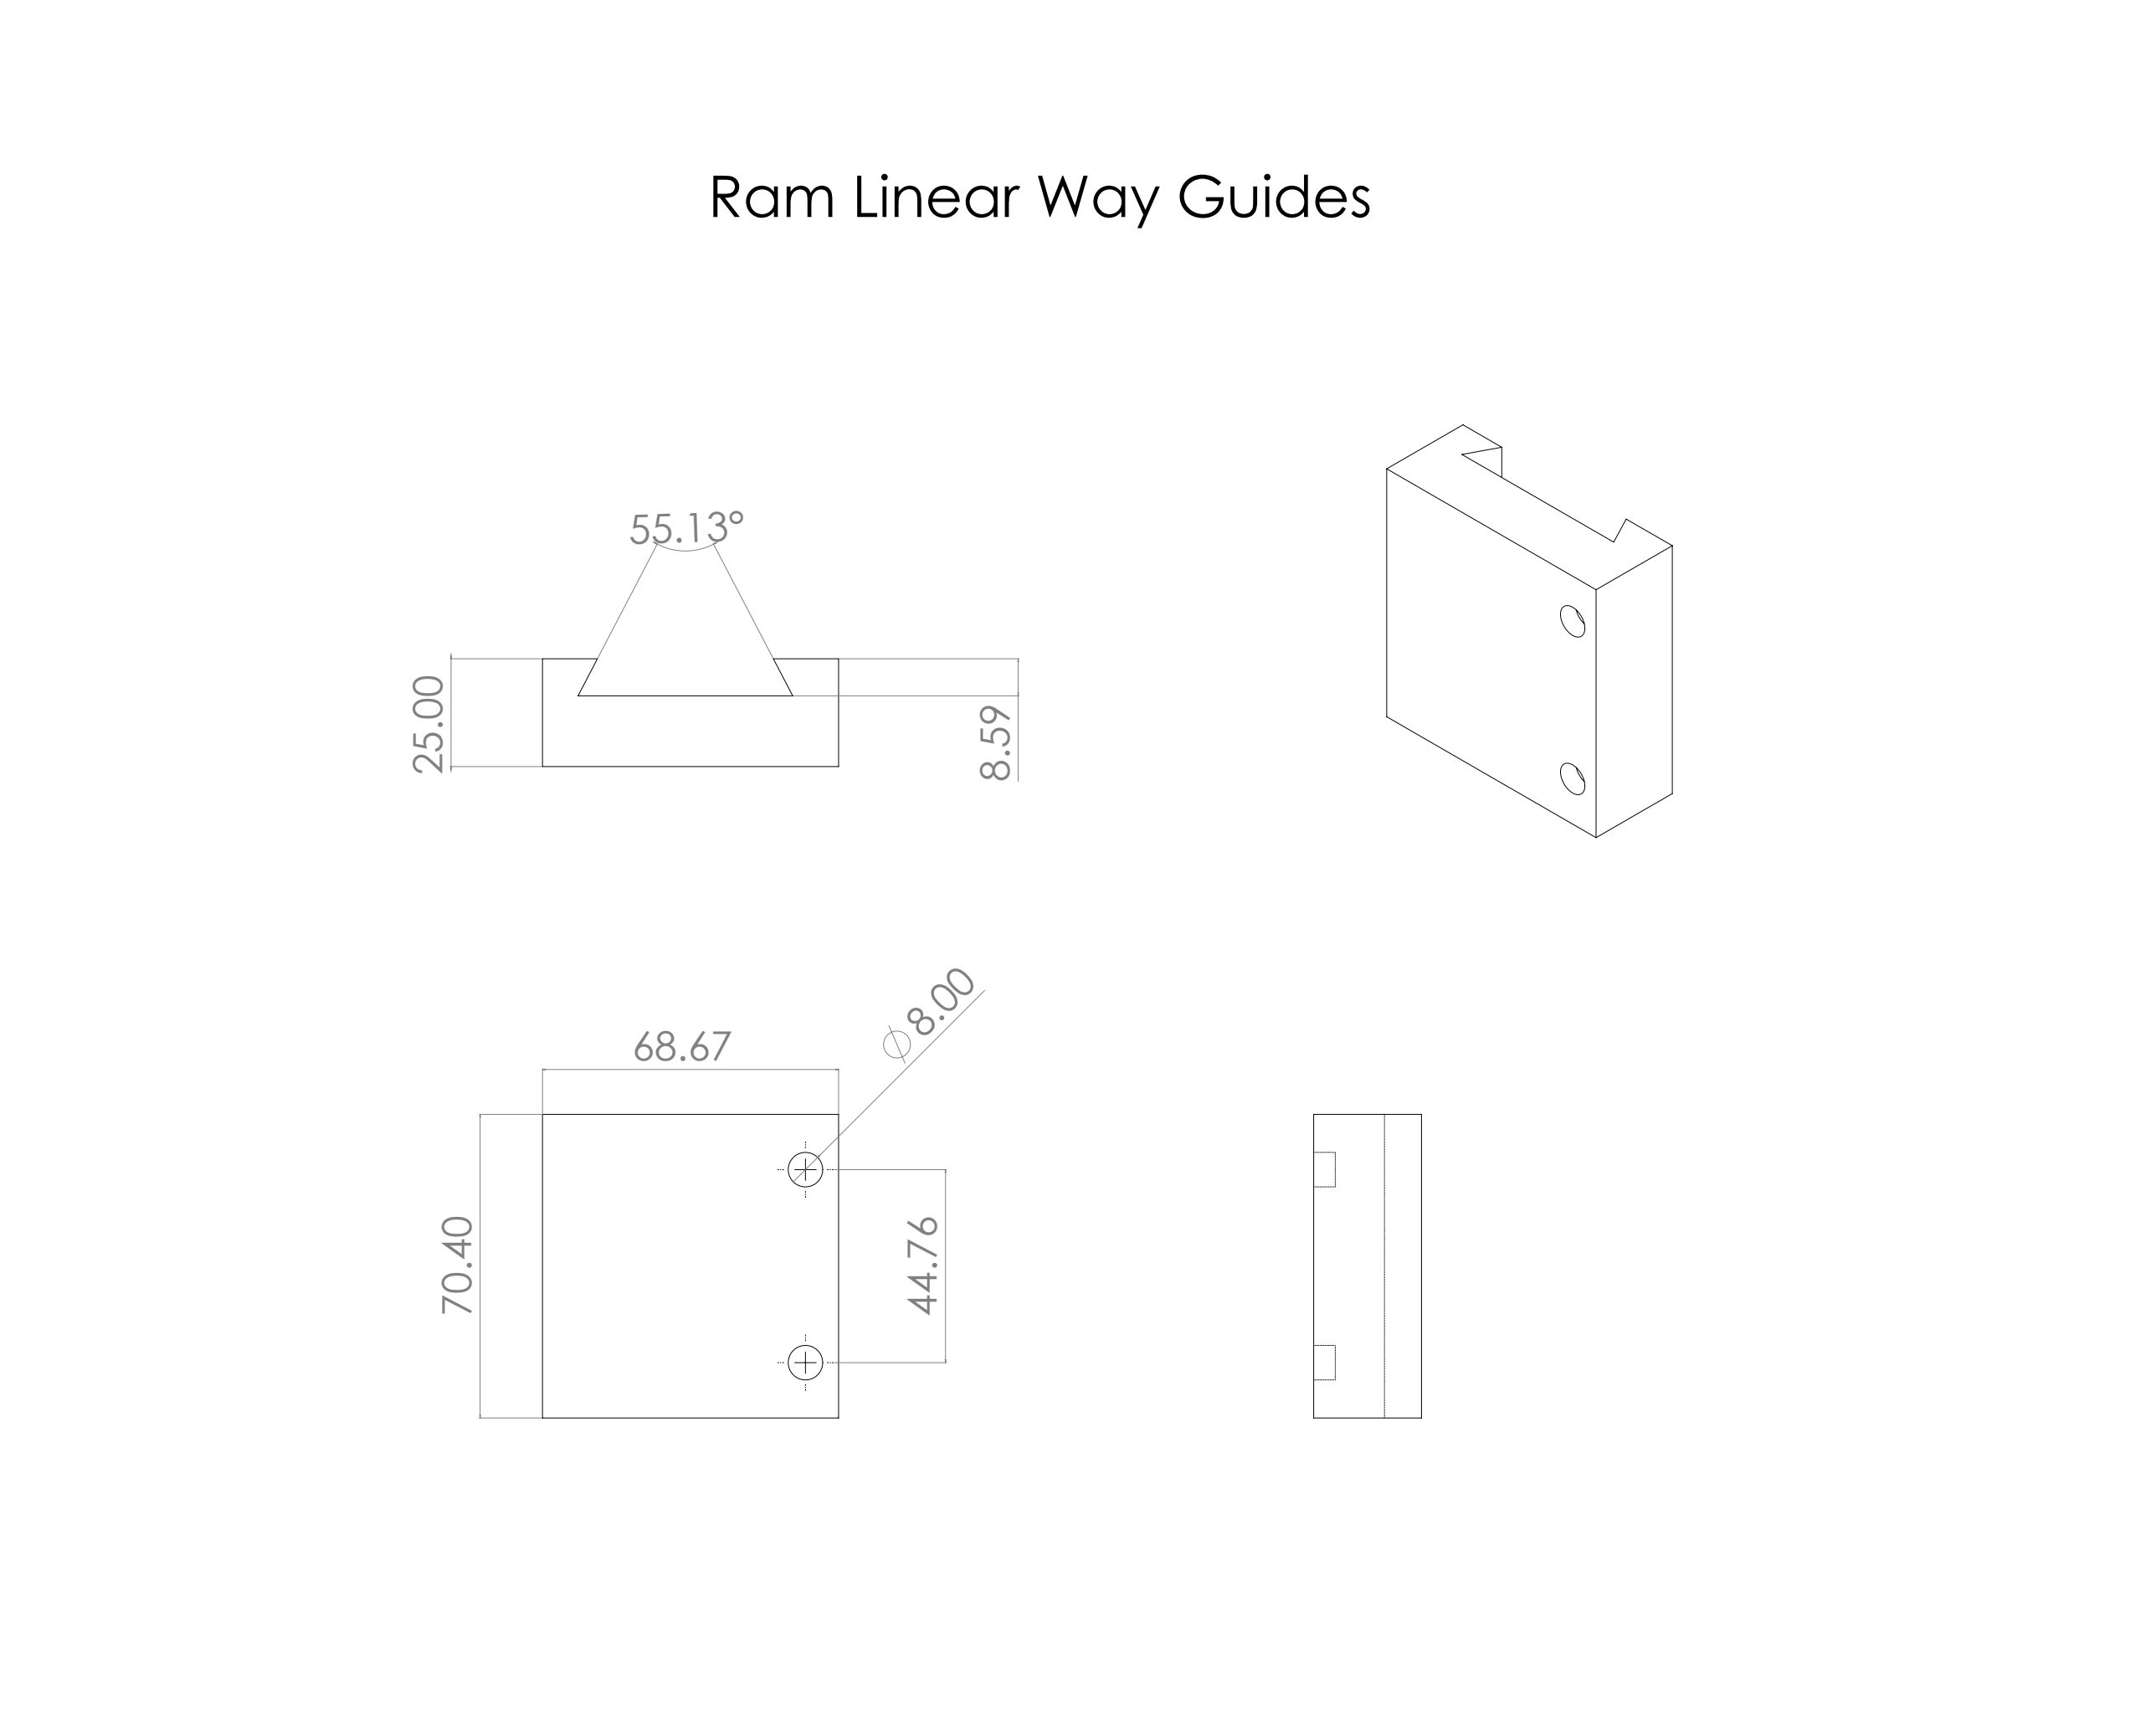
ISO-10303-21;
HEADER;
FILE_DESCRIPTION (('STEP AP214'),
    '1' );
FILE_NAME ('Ram Linear Way Guides.step',
    '2026-10-24T00:28:05',
    ( '' ),
    ( '' ),
    'SwSTEP 2.0',
    'SolidWorks 2025',
    '' );
FILE_SCHEMA (( 'AUTOMOTIVE_DESIGN' ));
ENDSEC;

DATA;
#156=CARTESIAN_POINT ( 'NONE',  ( -54.57497958038185004, 160.1716627696692683, 49.99999999999999289 ) ) ;
#191=ORIENTED_EDGE ( 'NONE', *, *, #19278, .F. ) ;
#197=DIRECTION ( 'NONE',  ( 0.000000000000000000, 0.000000000000000000, 1.000000000000000000 ) ) ;
#212=ORIENTED_EDGE ( 'NONE', *, *, #19326, .T. ) ;
#251=AXIS2_PLACEMENT_3D ( 'NONE', #16100, #3221, #14485 ) ;
#280=VECTOR ( 'NONE', #18343, 1000.000000000000000 ) ;
#332=DIRECTION ( 'NONE',  ( 0.000000000000000000, -0.000000000000000000, -1.000000000000000000 ) ) ;
#379=CARTESIAN_POINT ( 'NONE',  ( 6.416697501590670427, 172.9933428177121471, 45.00000000000000000 ) ) ;
#423=DIRECTION ( 'NONE',  ( 1.000000000000000000, 0.000000000000000000, -0.000000000000000000 ) ) ;
#438=DIRECTION ( 'NONE',  ( 0.000000000000000000, -1.000000000000000000, 0.000000000000000000 ) ) ;
#473=ORIENTED_EDGE ( 'NONE', *, *, #19536, .T. ) ;
#543=CARTESIAN_POINT ( 'NONE',  ( 10.41669750159067220, 217.7548513357008630, 45.00000000000000000 ) ) ;
#617=CARTESIAN_POINT ( 'NONE',  ( 6.416697501590670427, 172.9933428177121471, 49.99999999999999289 ) ) ;
#696=DIRECTION ( 'NONE',  ( 1.000000000000000000, 0.000000000000000000, 0.000000000000000000 ) ) ;
#718=( GEOMETRIC_REPRESENTATION_CONTEXT ( 3 ) GLOBAL_UNCERTAINTY_ASSIGNED_CONTEXT ( ( #1876 ) ) GLOBAL_UNIT_ASSIGNED_CONTEXT ( ( #11259, #6284, #3052 ) ) REPRESENTATION_CONTEXT ( 'NONE', 'WORKASPACE' ) );
#722=DIRECTION ( 'NONE',  ( 1.000000000000000000, 0.000000000000000000, 0.000000000000000000 ) ) ;
#751=CARTESIAN_POINT ( 'NONE',  ( 14.09825962131072785, 160.1716627696692683, 49.99999999999999289 ) ) ;
#808=CARTESIAN_POINT ( 'NONE',  ( 0.000000000000000000, 0.000000000000000000, 0.000000000000000000 ) ) ;
#884=PLANE ( 'NONE',  #19670 ) ;
#899=LINE ( 'NONE', #11030, #10091 ) ;
#918=PLANE ( 'NONE',  #7806 ) ;
#925=ORIENTED_EDGE ( 'NONE', *, *, #2214, .F. ) ;
#941=VECTOR ( 'NONE', #20908, 1000.000000000000000 ) ;
#965=PRODUCT_DEFINITION_SHAPE ( 'NONE', 'NONE',  #5449 ) ;
#976=ADVANCED_FACE ( 'NONE', ( #10029 ), #11976, .T. ) ;
#984=VERTEX_POINT ( 'NONE', #12082 ) ;
#1000=EDGE_CURVE ( 'NONE', #12300, #2829, #19044, .T. ) ;
#1005=DIRECTION ( 'NONE',  ( -1.000000000000000000, 0.000000000000000000, 0.000000000000000000 ) ) ;
#1044=DIRECTION ( 'NONE',  ( 0.000000000000000000, 0.000000000000000000, 1.000000000000000000 ) ) ;
#1053=CARTESIAN_POINT ( 'NONE',  ( -46.31968306282883674, 160.1716627696692683, 33.59072564020503648 ) ) ;
#1085=DIRECTION ( 'NONE',  ( -0.000000000000000000, -0.000000000000000000, 1.000000000000000000 ) ) ;
#1183=CARTESIAN_POINT ( 'NONE',  ( -41.83569717483972994, 303.6587712403113528, 25.00000000000000000 ) ) ;
#1274=VECTOR ( 'NONE', #21065, 1000.000000000000000 ) ;
#1308=CARTESIAN_POINT ( 'NONE',  ( 14.09825962131072785, 303.6587712403113528, 49.99999999999999289 ) ) ;
#1363=EDGE_LOOP ( 'NONE', ( #16478, #925, #12624, #3143 ) ) ;
#1437=CARTESIAN_POINT ( 'NONE',  ( 14.09825962131072785, 230.5765313837437418, 25.00000000000000000 ) ) ;
#1510=FACE_OUTER_BOUND ( 'NONE', #9710, .T. ) ;
#1527=LINE ( 'NONE', #9832, #3202 ) ;
#1544=CARTESIAN_POINT ( 'NONE',  ( 3.458603197740078627, 160.1716627696692683, 33.59072564020503648 ) ) ;
#1650=CARTESIAN_POINT ( 'NONE',  ( 6.416697501590670427, 217.7548513357008630, 49.99999999999999289 ) ) ;
#1668=LINE ( 'NONE', #2964, #11883 ) ;
#1698=ORIENTED_EDGE ( 'NONE', *, *, #13300, .F. ) ;
#1707=DIRECTION ( 'NONE',  ( 1.000000000000000000, 0.000000000000000000, 0.000000000000000000 ) ) ;
#1774=ORIENTED_EDGE ( 'NONE', *, *, #5730, .T. ) ;
#1777=LINE ( 'NONE', #19930, #14643 ) ;
#1778=ORIENTED_EDGE ( 'NONE', *, *, #18591, .F. ) ;
#1854=ORIENTED_EDGE ( 'NONE', *, *, #18917, .F. ) ;
#1856=ORIENTED_EDGE ( 'NONE', *, *, #19326, .F. ) ;
#1869=FACE_OUTER_BOUND ( 'NONE', #4529, .T. ) ;
#1876=UNCERTAINTY_MEASURE_WITH_UNIT (LENGTH_MEASURE( 1.000000000000000082E-05 ), #11259, 'distance_accuracy_value', 'NONE');
#1898=PLANE ( 'NONE',  #3083 ) ;
#2153=CYLINDRICAL_SURFACE ( 'NONE', #9746, 4.000000000000001776 ) ;
#2162=CIRCLE ( 'NONE', #7675, 4.000000000000001776 ) ;
#2214=EDGE_CURVE ( 'NONE', #17585, #2675, #8464, .T. ) ;
#2350=ORIENTED_EDGE ( 'NONE', *, *, #6167, .F. ) ;
#2386=DIRECTION ( 'NONE',  ( -0.000000000000000000, 0.000000000000000000, -1.000000000000000000 ) ) ;
#2394=DIRECTION ( 'NONE',  ( -1.000000000000000000, 0.000000000000000000, 0.000000000000000000 ) ) ;
#2419=DIRECTION ( 'NONE',  ( 0.000000000000000000, 0.000000000000000000, 1.000000000000000000 ) ) ;
#2535=VERTEX_POINT ( 'NONE', #10356 ) ;
#2564=AXIS2_PLACEMENT_3D ( 'NONE', #7882, #9824, #19676 ) ;
#2607=LINE ( 'NONE', #5840, #13238 ) ;
#2631=EDGE_CURVE ( 'NONE', #17585, #2829, #14280, .T. ) ;
#2675=VERTEX_POINT ( 'NONE', #20431 ) ;
#2704=DIRECTION ( 'NONE',  ( -1.000000000000000000, 0.000000000000000000, -0.000000000000000000 ) ) ;
#2721=VERTEX_POINT ( 'NONE', #751 ) ;
#2741=CARTESIAN_POINT ( 'NONE',  ( 2.416697501590669095, 172.9933428177121471, 49.99999999999999289 ) ) ;
#2751=ADVANCED_BREP_SHAPE_REPRESENTATION ( '', ( #19141, #12794 ), #718 ) ;
#2782=EDGE_LOOP ( 'NONE', ( #14261, #6010, #20550, #14725, #8206, #13930, #5554, #2865 ) ) ;
#2829=VERTEX_POINT ( 'NONE', #9157 ) ;
#2865=ORIENTED_EDGE ( 'NONE', *, *, #8030, .T. ) ;
#2910=VECTOR ( 'NONE', #1085, 1000.000000000000000 ) ;
#2964=CARTESIAN_POINT ( 'NONE',  ( 10.41669750159067220, 172.9933428177121471, 45.00000000000000000 ) ) ;
#3016=ORIENTED_EDGE ( 'NONE', *, *, #19278, .T. ) ;
#3052=( NAMED_UNIT ( * ) SI_UNIT ( $, .STERADIAN. ) SOLID_ANGLE_UNIT ( ) );
#3083=AXIS2_PLACEMENT_3D ( 'NONE', #379, #13571, #5328 ) ;
#3111=CARTESIAN_POINT ( 'NONE',  ( 2.416697501590669095, 217.7548513357008630, 49.99999999999999289 ) ) ;
#3121=ORIENTED_EDGE ( 'NONE', *, *, #16587, .F. ) ;
#3143=ORIENTED_EDGE ( 'NONE', *, *, #19941, .T. ) ;
#3150=EDGE_CURVE ( 'NONE', #16453, #6197, #1668, .T. ) ;
#3192=CARTESIAN_POINT ( 'NONE',  ( -54.57497958038185004, 230.5765313837437418, 49.99999999999999289 ) ) ;
#3198=EDGE_LOOP ( 'NONE', ( #21307, #15771, #9946, #212 ) ) ;
#3202=VECTOR ( 'NONE', #7993, 1000.000000000000000 ) ;
#3221=DIRECTION ( 'NONE',  ( -0.000000000000000000, -0.000000000000000000, 1.000000000000000000 ) ) ;
#3266=DIRECTION ( 'NONE',  ( -1.000000000000000000, 0.000000000000000000, 2.775557561562891844E-16 ) ) ;
#3364=CARTESIAN_POINT ( 'NONE',  ( -46.31968306282883674, 303.6587712403113528, 33.59072564020503648 ) ) ;
#3553=CARTESIAN_POINT ( 'NONE',  ( -41.83569717483972994, 303.6587712403113528, 25.00000000000000000 ) ) ;
#3716=EDGE_CURVE ( 'NONE', #6455, #20328, #899, .T. ) ;
#3717=VECTOR ( 'NONE', #20320, 1000.000000000000000 ) ;
#3750=ORIENTED_EDGE ( 'NONE', *, *, #16376, .T. ) ;
#3791=LINE ( 'NONE', #10277, #14282 ) ;
#3862=DIRECTION ( 'NONE',  ( 1.000000000000000000, 0.000000000000000000, 0.000000000000000000 ) ) ;
#3910=AXIS2_PLACEMENT_3D ( 'NONE', #617, #7181, #722 ) ;
#3927=EDGE_CURVE ( 'NONE', #20838, #9623, #1527, .T. ) ;
#3934=ORIENTED_EDGE ( 'NONE', *, *, #19941, .F. ) ;
#3969=CARTESIAN_POINT ( 'NONE',  ( -54.57497958038185715, 230.5765313837437418, 25.00000000000000000 ) ) ;
#4029=ADVANCED_FACE ( 'NONE', ( #20212 ), #2153, .F. ) ;
#4041=ORIENTED_EDGE ( 'NONE', *, *, #13300, .T. ) ;
#4089=CARTESIAN_POINT ( 'NONE',  ( 10.41669750159067220, 217.7548513357008630, 45.00000000000000000 ) ) ;
#4096=CARTESIAN_POINT ( 'NONE',  ( -54.57497958038185715, 303.6587712403113528, 25.00000000000000000 ) ) ;
#4162=DIRECTION ( 'NONE',  ( -0.000000000000000000, -0.000000000000000000, 1.000000000000000000 ) ) ;
#4200=AXIS2_PLACEMENT_3D ( 'NONE', #4096, #5933, #2704 ) ;
#4268=ORIENTED_EDGE ( 'NONE', *, *, #15151, .T. ) ;
#4273=CARTESIAN_POINT ( 'NONE',  ( -54.57497958038185715, 230.5765313837437418, 25.00000000000000000 ) ) ;
#4277=CARTESIAN_POINT ( 'NONE',  ( 14.09825962131072785, 160.1716627696692683, 25.00000000000000000 ) ) ;
#4340=ORIENTED_EDGE ( 'NONE', *, *, #20691, .T. ) ;
#4382=CARTESIAN_POINT ( 'NONE',  ( 6.416697501590670427, 172.9933428177121471, 45.00000000000000000 ) ) ;
#4436=CARTESIAN_POINT ( 'NONE',  ( -54.57497958038185004, 303.6587712403113528, 49.99999999999999289 ) ) ;
#4529=EDGE_LOOP ( 'NONE', ( #16668, #4268 ) ) ;
#4702=ORIENTED_EDGE ( 'NONE', *, *, #16376, .F. ) ;
#4717=( LENGTH_UNIT ( ) NAMED_UNIT ( * ) SI_UNIT ( .MILLI., .METRE. ) );
#4755=VERTEX_POINT ( 'NONE', #3192 ) ;
#4768=PLANE ( 'NONE',  #10337 ) ;
#4794=PLANE ( 'NONE',  #18083 ) ;
#4858=UNCERTAINTY_MEASURE_WITH_UNIT (LENGTH_MEASURE( 1.000000000000000082E-05 ), #4717, 'distance_accuracy_value', 'NONE');
#4865=DIRECTION ( 'NONE',  ( -1.000000000000000000, 0.000000000000000000, 0.000000000000000000 ) ) ;
#5079=CARTESIAN_POINT ( 'NONE',  ( 6.416697501590670427, 172.9933428177121471, 45.00000000000000000 ) ) ;
#5081=ORIENTED_EDGE ( 'NONE', *, *, #3716, .F. ) ;
#5099=PRODUCT_DEFINITION_CONTEXT ( 'detailed design', #20777, 'design' ) ;
#5197=DIRECTION ( 'NONE',  ( 0.000000000000000000, 0.000000000000000000, 1.000000000000000000 ) ) ;
#5267=VERTEX_POINT ( 'NONE', #2741 ) ;
#5287=CARTESIAN_POINT ( 'NONE',  ( -1.025382690249031503, 230.5765313837437418, 25.00000000000000000 ) ) ;
#5328=DIRECTION ( 'NONE',  ( -1.000000000000000000, 0.000000000000000000, 0.000000000000000000 ) ) ;
#5348=EDGE_LOOP ( 'NONE', ( #1856, #19473 ) ) ;
#5449=PRODUCT_DEFINITION ( 'UNKNOWN', '', #17987, #5099 ) ;
#5474=ORIENTED_EDGE ( 'NONE', *, *, #6268, .T. ) ;
#5482=DIRECTION ( 'NONE',  ( 0.8865057725575725689, 0.000000000000000000, 0.4627175328665443232 ) ) ;
#5514=PLANE ( 'NONE',  #18980 ) ;
#5528=ORIENTED_EDGE ( 'NONE', *, *, #11209, .T. ) ;
#5554=ORIENTED_EDGE ( 'NONE', *, *, #6229, .T. ) ;
#5582=ORIENTED_EDGE ( 'NONE', *, *, #17769, .T. ) ;
#5730=EDGE_CURVE ( 'NONE', #4755, #15709, #12562, .T. ) ;
#5819=EDGE_LOOP ( 'NONE', ( #17219, #13840, #8937, #1698 ) ) ;
#5840=CARTESIAN_POINT ( 'NONE',  ( -46.31968306282883674, 160.1716627696692683, 33.59072564020503648 ) ) ;
#5867=DIRECTION ( 'NONE',  ( -0.4627175328665442677, 0.000000000000000000, -0.8865057725575725689 ) ) ;
#5891=CYLINDRICAL_SURFACE ( 'NONE', #10934, 4.000000000000001776 ) ;
#5933=DIRECTION ( 'NONE',  ( 0.000000000000000000, 0.000000000000000000, -1.000000000000000000 ) ) ;
#5975=CIRCLE ( 'NONE', #19457, 4.000000000000001776 ) ;
#6010=ORIENTED_EDGE ( 'NONE', *, *, #7435, .T. ) ;
#6073=CARTESIAN_POINT ( 'NONE',  ( -54.57497958038185004, 230.5765313837437418, 49.99999999999999289 ) ) ;
#6113=ORIENTED_EDGE ( 'NONE', *, *, #13198, .T. ) ;
#6167=EDGE_CURVE ( 'NONE', #15709, #20838, #6614, .T. ) ;
#6197=VERTEX_POINT ( 'NONE', #6830 ) ;
#6214=CARTESIAN_POINT ( 'NONE',  ( -41.83569717483972994, 230.5765313837437418, 25.00000000000000000 ) ) ;
#6229=EDGE_CURVE ( 'NONE', #2535, #7734, #1777, .T. ) ;
#6268=EDGE_CURVE ( 'NONE', #2721, #15709, #7247, .T. ) ;
#6284=( NAMED_UNIT ( * ) PLANE_ANGLE_UNIT ( ) SI_UNIT ( $, .RADIAN. ) );
#6329=ORIENTED_EDGE ( 'NONE', *, *, #9299, .T. ) ;
#6411=FACE_OUTER_BOUND ( 'NONE', #7242, .T. ) ;
#6434=EDGE_CURVE ( 'NONE', #16453, #10176, #5975, .T. ) ;
#6455=VERTEX_POINT ( 'NONE', #5287 ) ;
#6493=DIRECTION ( 'NONE',  ( 1.000000000000000000, 0.000000000000000000, 0.000000000000000000 ) ) ;
#6525=VECTOR ( 'NONE', #14000, 1000.000000000000114 ) ;
#6614=LINE ( 'NONE', #156, #11507 ) ;
#6671=VECTOR ( 'NONE', #7077, 1000.000000000000000 ) ;
#6796=AXIS2_PLACEMENT_3D ( 'NONE', #10408, #18526, #13781 ) ;
#6817=CARTESIAN_POINT ( 'NONE',  ( 14.09825962131072785, 160.1716627696692683, 25.00000000000000000 ) ) ;
#6830=CARTESIAN_POINT ( 'NONE',  ( 10.41669750159067220, 172.9933428177121471, 49.99999999999999289 ) ) ;
#6996=ORIENTED_EDGE ( 'NONE', *, *, #17769, .F. ) ;
#6997=DIRECTION ( 'NONE',  ( 0.4627175328665442677, 0.000000000000000000, -0.8865057725575724579 ) ) ;
#7004=CARTESIAN_POINT ( 'NONE',  ( 20.42502041961813930, 230.5765313837437418, 60.00000000000000000 ) ) ;
#7006=VECTOR ( 'NONE', #19540, 1000.000000000000000 ) ;
#7021=CIRCLE ( 'NONE', #9096, 4.000000000000001776 ) ;
#7039=EDGE_LOOP ( 'NONE', ( #11206, #3750 ) ) ;
#7077=DIRECTION ( 'NONE',  ( 0.000000000000000000, -1.000000000000000000, 0.000000000000000000 ) ) ;
#7181=DIRECTION ( 'NONE',  ( 0.000000000000000000, 0.000000000000000000, 1.000000000000000000 ) ) ;
#7242=EDGE_LOOP ( 'NONE', ( #17088, #4041, #18357, #13154 ) ) ;
#7247=LINE ( 'NONE', #18826, #12567 ) ;
#7334=VERTEX_POINT ( 'NONE', #20095 ) ;
#7372=CARTESIAN_POINT ( 'NONE',  ( -41.83569717483972994, 160.1716627696692683, 25.00000000000000000 ) ) ;
#7435=EDGE_CURVE ( 'NONE', #4755, #984, #17066, .T. ) ;
#7478=CARTESIAN_POINT ( 'NONE',  ( 10.41669750159067220, 172.9933428177121471, 45.00000000000000000 ) ) ;
#7589=CARTESIAN_POINT ( 'NONE',  ( 3.458603197740078627, 160.1716627696692683, 33.59072564020503648 ) ) ;
#7660=FACE_OUTER_BOUND ( 'NONE', #12569, .T. ) ;
#7675=AXIS2_PLACEMENT_3D ( 'NONE', #19973, #197, #1707 ) ;
#7734=VERTEX_POINT ( 'NONE', #6214 ) ;
#7775=DIRECTION ( 'NONE',  ( 0.000000000000000000, -1.000000000000000000, 0.000000000000000000 ) ) ;
#7806=AXIS2_PLACEMENT_3D ( 'NONE', #14109, #14217, #20804 ) ;
#7847=AXIS2_PLACEMENT_3D ( 'NONE', #17108, #8867, #15067 ) ;
#7882=CARTESIAN_POINT ( 'NONE',  ( 6.416697501590670427, 217.7548513357008630, 45.00000000000000000 ) ) ;
#7993=DIRECTION ( 'NONE',  ( 1.000000000000000000, 0.000000000000000000, 0.000000000000000000 ) ) ;
#8030=EDGE_CURVE ( 'NONE', #7734, #8775, #15564, .T. ) ;
#8084=DIRECTION ( 'NONE',  ( -0.000000000000000000, -0.000000000000000000, 1.000000000000000000 ) ) ;
#8173=LINE ( 'NONE', #1183, #1274 ) ;
#8204=ORIENTED_EDGE ( 'NONE', *, *, #3927, .F. ) ;
#8206=ORIENTED_EDGE ( 'NONE', *, *, #3716, .T. ) ;
#8209=EDGE_LOOP ( 'NONE', ( #17696, #10470, #16403, #6996 ) ) ;
#8401=CIRCLE ( 'NONE', #3910, 4.000000000000001776 ) ;
#8464=CIRCLE ( 'NONE', #2564, 4.000000000000001776 ) ;
#8690=DIRECTION ( 'NONE',  ( 0.000000000000000000, -1.000000000000000000, 0.000000000000000000 ) ) ;
#8766=PLANE ( 'NONE',  #7847 ) ;
#8775=VERTEX_POINT ( 'NONE', #4273 ) ;
#8789=FACE_OUTER_BOUND ( 'NONE', #7039, .T. ) ;
#8867=DIRECTION ( 'NONE',  ( 0.000000000000000000, 0.000000000000000000, 1.000000000000000000 ) ) ;
#8937=ORIENTED_EDGE ( 'NONE', *, *, #20917, .F. ) ;
#9096=AXIS2_PLACEMENT_3D ( 'NONE', #1650, #10061, #6493 ) ;
#9130=CARTESIAN_POINT ( 'NONE',  ( 2.416697501590669095, 217.7548513357008630, 45.00000000000000000 ) ) ;
#9157=CARTESIAN_POINT ( 'NONE',  ( 10.41669750159067220, 217.7548513357008630, 49.99999999999999289 ) ) ;
#9175=ADVANCED_FACE ( 'NONE', ( #8789 ), #1898, .F. ) ;
#9241=CARTESIAN_POINT ( 'NONE',  ( 6.416697501590670427, 217.7548513357008630, 45.00000000000000000 ) ) ;
#9243=CARTESIAN_POINT ( 'NONE',  ( -54.57497958038185715, 160.1716627696692683, 25.00000000000000000 ) ) ;
#9269=VECTOR ( 'NONE', #16864, 1000.000000000000000 ) ;
#9292=FACE_OUTER_BOUND ( 'NONE', #5819, .T. ) ;
#9299=EDGE_CURVE ( 'NONE', #9623, #12668, #17652, .T. ) ;
#9377=LINE ( 'NONE', #15013, #7006 ) ;
#9383=FACE_OUTER_BOUND ( 'NONE', #17142, .T. ) ;
#9457=LINE ( 'NONE', #9130, #14990 ) ;
#9558=ADVANCED_FACE ( 'NONE', ( #16465 ), #4768, .T. ) ;
#9574=CIRCLE ( 'NONE', #12344, 4.000000000000001776 ) ;
#9623=VERTEX_POINT ( 'NONE', #20339 ) ;
#9660=CARTESIAN_POINT ( 'NONE',  ( -1.025382690249029949, 303.6587712403113528, 25.00000000000000000 ) ) ;
#9704=ADVANCED_FACE ( 'NONE', ( #1869 ), #5514, .T. ) ;
#9710=EDGE_LOOP ( 'NONE', ( #18437, #473, #18248, #17350 ) ) ;
#9746=AXIS2_PLACEMENT_3D ( 'NONE', #12416, #13831, #14272 ) ;
#9809=LINE ( 'NONE', #16432, #13893 ) ;
#9824=DIRECTION ( 'NONE',  ( 0.000000000000000000, 0.000000000000000000, 1.000000000000000000 ) ) ;
#9832=CARTESIAN_POINT ( 'NONE',  ( -54.57497958038185715, 160.1716627696692683, 25.00000000000000000 ) ) ;
#9890=ORIENTED_EDGE ( 'NONE', *, *, #20917, .T. ) ;
#9929=ADVANCED_FACE ( 'NONE', ( #9292 ), #884, .T. ) ;
#9946=ORIENTED_EDGE ( 'NONE', *, *, #3150, .T. ) ;
#10029=FACE_OUTER_BOUND ( 'NONE', #8209, .T. ) ;
#10052=ADVANCED_FACE ( 'NONE', ( #17625 ), #21192, .T. ) ;
#10061=DIRECTION ( 'NONE',  ( 0.000000000000000000, 0.000000000000000000, 1.000000000000000000 ) ) ;
#10075=DIRECTION ( 'NONE',  ( 0.4627175328665443232, 0.000000000000000000, -0.8865057725575725689 ) ) ;
#10091=VECTOR ( 'NONE', #14200, 999.9999999999998863 ) ;
#10121=( GEOMETRIC_REPRESENTATION_CONTEXT ( 3 ) GLOBAL_UNCERTAINTY_ASSIGNED_CONTEXT ( ( #4858 ) ) GLOBAL_UNIT_ASSIGNED_CONTEXT ( ( #4717, #21269, #19641 ) ) REPRESENTATION_CONTEXT ( 'NONE', 'WORKASPACE' ) );
#10176=VERTEX_POINT ( 'NONE', #12869 ) ;
#10200=ADVANCED_FACE ( 'NONE', ( #1510 ), #11234, .F. ) ;
#10277=CARTESIAN_POINT ( 'NONE',  ( -46.31968306282883674, 230.5765313837437418, 33.59072564020503648 ) ) ;
#10303=CARTESIAN_POINT ( 'NONE',  ( -46.31968306282883674, 303.6587712403113528, 33.59072564020503648 ) ) ;
#10337=AXIS2_PLACEMENT_3D ( 'NONE', #11363, #3266, #11257 ) ;
#10353=CARTESIAN_POINT ( 'NONE',  ( 14.09825962131072785, 230.5765313837437418, 25.00000000000000000 ) ) ;
#10356=CARTESIAN_POINT ( 'NONE',  ( -46.31968306282883674, 230.5765313837437418, 33.59072564020503648 ) ) ;
#10408=CARTESIAN_POINT ( 'NONE',  ( 6.416697501590670427, 172.9933428177121471, 45.00000000000000000 ) ) ;
#10470=ORIENTED_EDGE ( 'NONE', *, *, #14529, .T. ) ;
#10488=ADVANCED_FACE ( 'NONE', ( #11463 ), #18062, .T. ) ;
#10691=CARTESIAN_POINT ( 'NONE',  ( 14.09825962131072785, 303.6587712403113528, 25.00000000000000000 ) ) ;
#10859=DIRECTION ( 'NONE',  ( 1.000000000000000000, 0.000000000000000000, 0.000000000000000000 ) ) ;
#10921=ORIENTED_EDGE ( 'NONE', *, *, #8030, .F. ) ;
#10927=ADVANCED_FACE ( 'NONE', ( #7660 ), #11009, .T. ) ;
#10934=AXIS2_PLACEMENT_3D ( 'NONE', #4382, #4162, #12387 ) ;
#11009=PLANE ( 'NONE',  #4200 ) ;
#11030=CARTESIAN_POINT ( 'NONE',  ( 3.458603197740078627, 230.5765313837437418, 33.59072564020503648 ) ) ;
#11043=SHAPE_REPRESENTATION_RELATIONSHIP ( 'NONE' , 'NONE' ,  #15840, #2751 ) ;
#11045=DIRECTION ( 'NONE',  ( 2.775557561562891844E-16, 0.000000000000000000, 1.000000000000000000 ) ) ;
#11077=VECTOR ( 'NONE', #7775, 1000.000000000000000 ) ;
#11082=AXIS2_PLACEMENT_3D ( 'NONE', #3553, #5482, #6997 ) ;
#11160=LINE ( 'NONE', #7589, #14058 ) ;
#11206=ORIENTED_EDGE ( 'NONE', *, *, #6434, .T. ) ;
#11209=EDGE_CURVE ( 'NONE', #7334, #20009, #9809, .T. ) ;
#11219=CYLINDRICAL_SURFACE ( 'NONE', #251, 4.000000000000001776 ) ;
#11234=CYLINDRICAL_SURFACE ( 'NONE', #18631, 4.000000000000001776 ) ;
#11257=DIRECTION ( 'NONE',  ( 2.775557561562891844E-16, 0.000000000000000000, 1.000000000000000000 ) ) ;
#11259=( LENGTH_UNIT ( ) NAMED_UNIT ( * ) SI_UNIT ( .MILLI., .METRE. ) );
#11363=CARTESIAN_POINT ( 'NONE',  ( -54.57497958038185004, 303.6587712403113528, 49.99999999999999289 ) ) ;
#11390=DIRECTION ( 'NONE',  ( -1.000000000000000000, 0.000000000000000000, -0.000000000000000000 ) ) ;
#11417=LINE ( 'NONE', #19971, #280 ) ;
#11458=DIRECTION ( 'NONE',  ( 0.000000000000000000, 0.000000000000000000, 1.000000000000000000 ) ) ;
#11463=FACE_OUTER_BOUND ( 'NONE', #16159, .T. ) ;
#11499=SHAPE_DEFINITION_REPRESENTATION ( #965, #15840 ) ;
#11507=VECTOR ( 'NONE', #18509, 1000.000000000000000 ) ;
#11512=VECTOR ( 'NONE', #19466, 1000.000000000000000 ) ;
#11522=VECTOR ( 'NONE', #423, 1000.000000000000000 ) ;
#11643=VECTOR ( 'NONE', #18764, 1000.000000000000000 ) ;
#11883=VECTOR ( 'NONE', #13345, 1000.000000000000000 ) ;
#11955=LINE ( 'NONE', #15431, #6671 ) ;
#11961=AXIS2_PLACEMENT_3D ( 'NONE', #7004, #438, #332 ) ;
#11976=PLANE ( 'NONE',  #11082 ) ;
#11978=VECTOR ( 'NONE', #12929, 1000.000000000000000 ) ;
#12008=DIRECTION ( 'NONE',  ( 1.000000000000000000, 0.000000000000000000, -0.000000000000000000 ) ) ;
#12082=CARTESIAN_POINT ( 'NONE',  ( 14.09825962131072785, 230.5765313837437418, 49.99999999999999289 ) ) ;
#12093=LINE ( 'NONE', #10353, #3717 ) ;
#12097=CLOSED_SHELL ( 'NONE', ( #10200, #17932, #9558, #16893, #9929, #19732, #10052, #10488, #976, #10927, #13281, #17570, #15938, #9175, #4029, #9704 ) ) ;
#12176=LINE ( 'NONE', #4277, #19769 ) ;
#12177=CARTESIAN_POINT ( 'NONE',  ( -1.025382690249029949, 303.6587712403113528, 25.00000000000000000 ) ) ;
#12300=VERTEX_POINT ( 'NONE', #3111 ) ;
#12344=AXIS2_PLACEMENT_3D ( 'NONE', #9241, #1044, #10859 ) ;
#12387=DIRECTION ( 'NONE',  ( 1.000000000000000000, 0.000000000000000000, 0.000000000000000000 ) ) ;
#12416=CARTESIAN_POINT ( 'NONE',  ( 6.416697501590670427, 217.7548513357008630, 45.00000000000000000 ) ) ;
#12487=AXIS2_PLACEMENT_3D ( 'NONE', #16863, #18673, #3862 ) ;
#12562=LINE ( 'NONE', #4436, #11077 ) ;
#12567=VECTOR ( 'NONE', #1005, 1000.000000000000000 ) ;
#12569=EDGE_LOOP ( 'NONE', ( #10921, #5582, #8204, #14064 ) ) ;
#12624=ORIENTED_EDGE ( 'NONE', *, *, #2631, .T. ) ;
#12668=VERTEX_POINT ( 'NONE', #1053 ) ;
#12687=CARTESIAN_POINT ( 'NONE',  ( 14.09825962131072785, 303.6587712403113528, 25.00000000000000000 ) ) ;
#12761=CARTESIAN_POINT ( 'NONE',  ( 3.458603197740078627, 303.6587712403113528, 33.59072564020503648 ) ) ;
#12794=AXIS2_PLACEMENT_3D ( 'NONE', #808, #2419, #696 ) ;
#12869=CARTESIAN_POINT ( 'NONE',  ( 2.416697501590669095, 172.9933428177121471, 45.00000000000000000 ) ) ;
#12882=ORIENTED_EDGE ( 'NONE', *, *, #6167, .T. ) ;
#12929=DIRECTION ( 'NONE',  ( 0.000000000000000000, -1.000000000000000000, 0.000000000000000000 ) ) ;
#12983=ORIENTED_EDGE ( 'NONE', *, *, #13198, .F. ) ;
#13154=ORIENTED_EDGE ( 'NONE', *, *, #15729, .F. ) ;
#13198=EDGE_CURVE ( 'NONE', #18325, #7334, #11160, .T. ) ;
#13238=VECTOR ( 'NONE', #17527, 1000.000000000000000 ) ;
#13281=ADVANCED_FACE ( 'NONE', ( #15732 ), #918, .T. ) ;
#13300=EDGE_CURVE ( 'NONE', #16828, #20009, #15941, .T. ) ;
#13304=CARTESIAN_POINT ( 'NONE',  ( -54.57497958038185004, 160.1716627696692683, 49.99999999999999289 ) ) ;
#13317=ORIENTED_EDGE ( 'NONE', *, *, #14529, .F. ) ;
#13320=DIRECTION ( 'NONE',  ( -1.000000000000000000, 0.000000000000000000, -0.000000000000000000 ) ) ;
#13345=DIRECTION ( 'NONE',  ( -0.000000000000000000, -0.000000000000000000, 1.000000000000000000 ) ) ;
#13379=VECTOR ( 'NONE', #8690, 1000.000000000000000 ) ;
#13547=FACE_BOUND ( 'NONE', #20769, .T. ) ;
#13558=EDGE_LOOP ( 'NONE', ( #3121, #15394, #2350, #18055 ) ) ;
#13571=DIRECTION ( 'NONE',  ( -0.000000000000000000, 0.000000000000000000, -1.000000000000000000 ) ) ;
#13601=STYLED_ITEM('',(#21428),#19141);
#13646=CARTESIAN_POINT ( 'NONE',  ( 6.416697501590670427, 217.7548513357008630, 45.00000000000000000 ) ) ;
#13692=ORIENTED_EDGE ( 'NONE', *, *, #7435, .F. ) ;
#13781=DIRECTION ( 'NONE',  ( -1.000000000000000000, 0.000000000000000000, 0.000000000000000000 ) ) ;
#13831=DIRECTION ( 'NONE',  ( -0.000000000000000000, -0.000000000000000000, 1.000000000000000000 ) ) ;
#13840=ORIENTED_EDGE ( 'NONE', *, *, #18917, .T. ) ;
#13864=FACE_OUTER_BOUND ( 'NONE', #16129, .T. ) ;
#13874=AXIS2_PLACEMENT_3D ( 'NONE', #3364, #16245, #13320 ) ;
#13893=VECTOR ( 'NONE', #16537, 1000.000000000000000 ) ;
#13930=ORIENTED_EDGE ( 'NONE', *, *, #18591, .T. ) ;
#14000=DIRECTION ( 'NONE',  ( -0.4627175328665442677, 0.000000000000000000, 0.8865057725575725689 ) ) ;
#14058=VECTOR ( 'NONE', #5867, 1000.000000000000114 ) ;
#14064=ORIENTED_EDGE ( 'NONE', *, *, #16052, .F. ) ;
#14109=CARTESIAN_POINT ( 'NONE',  ( 0.000000000000000000, 160.1716627696692683, 0.000000000000000000 ) ) ;
#14200=DIRECTION ( 'NONE',  ( 0.4627175328665443232, 0.000000000000000000, 0.8865057725575725689 ) ) ;
#14217=DIRECTION ( 'NONE',  ( 0.000000000000000000, -1.000000000000000000, 0.000000000000000000 ) ) ;
#14261=ORIENTED_EDGE ( 'NONE', *, *, #16587, .T. ) ;
#14272=DIRECTION ( 'NONE',  ( 1.000000000000000000, 0.000000000000000000, 0.000000000000000000 ) ) ;
#14280=LINE ( 'NONE', #4089, #2910 ) ;
#14282=VECTOR ( 'NONE', #2394, 1000.000000000000000 ) ;
#14485=DIRECTION ( 'NONE',  ( 1.000000000000000000, 0.000000000000000000, 0.000000000000000000 ) ) ;
#14507=LINE ( 'NONE', #1308, #11512 ) ;
#14529=EDGE_CURVE ( 'NONE', #2535, #12668, #20271, .T. ) ;
#14620=ORIENTED_EDGE ( 'NONE', *, *, #15729, .T. ) ;
#14643=VECTOR ( 'NONE', #10075, 999.9999999999998863 ) ;
#14725=ORIENTED_EDGE ( 'NONE', *, *, #19149, .T. ) ;
#14792=EDGE_CURVE ( 'NONE', #10176, #5267, #11417, .T. ) ;
#14798=CARTESIAN_POINT ( 'NONE',  ( 3.458603197740078627, 230.5765313837437418, 33.59072564020503648 ) ) ;
#14820=CARTESIAN_POINT ( 'NONE',  ( 6.416697501590670427, 217.7548513357008630, 45.00000000000000000 ) ) ;
#14970=APPLICATION_CONTEXT ( 'automotive_design' ) ;
#14990=VECTOR ( 'NONE', #20929, 1000.000000000000000 ) ;
#15013=CARTESIAN_POINT ( 'NONE',  ( -1.025382690249029949, 230.5765313837437418, 25.00000000000000000 ) ) ;
#15067=DIRECTION ( 'NONE',  ( 1.000000000000000000, 0.000000000000000000, -0.000000000000000000 ) ) ;
#15151=EDGE_CURVE ( 'NONE', #2675, #17585, #9574, .T. ) ;
#15251=FACE_OUTER_BOUND ( 'NONE', #2782, .T. ) ;
#15280=FACE_BOUND ( 'NONE', #5348, .T. ) ;
#15394=ORIENTED_EDGE ( 'NONE', *, *, #16052, .T. ) ;
#15431=CARTESIAN_POINT ( 'NONE',  ( 3.458603197740078627, 303.6587712403113528, 33.59072564020503648 ) ) ;
#15564=LINE ( 'NONE', #3969, #9269 ) ;
#15709=VERTEX_POINT ( 'NONE', #13304 ) ;
#15729=EDGE_CURVE ( 'NONE', #6455, #7334, #20398, .T. ) ;
#15732=FACE_OUTER_BOUND ( 'NONE', #18009, .T. ) ;
#15771=ORIENTED_EDGE ( 'NONE', *, *, #6434, .F. ) ;
#15807=DIRECTION ( 'NONE',  ( 1.000000000000000000, 0.000000000000000000, -0.000000000000000000 ) ) ;
#15840=SHAPE_REPRESENTATION ( 'Ram Linear Way Guides', ( #12794 ), #718 ) ;
#15899=ORIENTED_EDGE ( 'NONE', *, *, #14792, .T. ) ;
#15938=ADVANCED_FACE ( 'NONE', ( #17684 ), #5891, .F. ) ;
#15941=LINE ( 'NONE', #12687, #941 ) ;
#16052=EDGE_CURVE ( 'NONE', #8775, #20838, #16395, .T. ) ;
#16100=CARTESIAN_POINT ( 'NONE',  ( 6.416697501590670427, 172.9933428177121471, 45.00000000000000000 ) ) ;
#16129=EDGE_LOOP ( 'NONE', ( #13692, #1774, #18755, #1854 ) ) ;
#16144=CIRCLE ( 'NONE', #6796, 4.000000000000001776 ) ;
#16159=EDGE_LOOP ( 'NONE', ( #1778, #3016, #18807, #13317 ) ) ;
#16245=DIRECTION ( 'NONE',  ( 0.000000000000000000, 0.000000000000000000, -1.000000000000000000 ) ) ;
#16376=EDGE_CURVE ( 'NONE', #10176, #16453, #16144, .T. ) ;
#16395=LINE ( 'NONE', #21356, #11978 ) ;
#16403=ORIENTED_EDGE ( 'NONE', *, *, #9299, .F. ) ;
#16432=CARTESIAN_POINT ( 'NONE',  ( -1.025382690249029949, 160.1716627696692683, 25.00000000000000000 ) ) ;
#16453=VERTEX_POINT ( 'NONE', #7478 ) ;
#16465=FACE_OUTER_BOUND ( 'NONE', #13558, .T. ) ;
#16478=ORIENTED_EDGE ( 'NONE', *, *, #19536, .F. ) ;
#16537=DIRECTION ( 'NONE',  ( 1.000000000000000000, 0.000000000000000000, 0.000000000000000000 ) ) ;
#16587=EDGE_CURVE ( 'NONE', #8775, #4755, #20802, .T. ) ;
#16597=PRODUCT_CONTEXT ( 'NONE', #14970, 'mechanical' ) ;
#16668=ORIENTED_EDGE ( 'NONE', *, *, #2214, .T. ) ;
#16697=ORIENTED_EDGE ( 'NONE', *, *, #3927, .T. ) ;
#16699=MECHANICAL_DESIGN_GEOMETRIC_PRESENTATION_REPRESENTATION('',(#13601),#10121);
#16828=VERTEX_POINT ( 'NONE', #1437 ) ;
#16863=CARTESIAN_POINT ( 'NONE',  ( 6.416697501590670427, 217.7548513357008630, 49.99999999999999289 ) ) ;
#16864=DIRECTION ( 'NONE',  ( -1.000000000000000000, 0.000000000000000000, 0.000000000000000000 ) ) ;
#16893=ADVANCED_FACE ( 'NONE', ( #13547, #15280, #13864 ), #8766, .T. ) ;
#17066=LINE ( 'NONE', #18245, #11522 ) ;
#17088=ORIENTED_EDGE ( 'NONE', *, *, #19149, .F. ) ;
#17108=CARTESIAN_POINT ( 'NONE',  ( 14.09825962131072785, 303.6587712403113528, 49.99999999999999289 ) ) ;
#17142=EDGE_LOOP ( 'NONE', ( #4702, #15899, #4340, #20567 ) ) ;
#17157=DIRECTION ( 'NONE',  ( 0.000000000000000000, 0.000000000000000000, 1.000000000000000000 ) ) ;
#17171=ORIENTED_EDGE ( 'NONE', *, *, #1000, .F. ) ;
#17219=ORIENTED_EDGE ( 'NONE', *, *, #17488, .F. ) ;
#17350=ORIENTED_EDGE ( 'NONE', *, *, #2631, .F. ) ;
#17488=EDGE_CURVE ( 'NONE', #984, #16828, #12093, .T. ) ;
#17527=DIRECTION ( 'NONE',  ( 1.000000000000000000, 0.000000000000000000, 0.000000000000000000 ) ) ;
#17570=ADVANCED_FACE ( 'NONE', ( #15251 ), #20215, .F. ) ;
#17585=VERTEX_POINT ( 'NONE', #543 ) ;
#17625=FACE_OUTER_BOUND ( 'NONE', #19556, .T. ) ;
#17652=LINE ( 'NONE', #7372, #6525 ) ;
#17684=FACE_OUTER_BOUND ( 'NONE', #3198, .T. ) ;
#17696=ORIENTED_EDGE ( 'NONE', *, *, #6229, .F. ) ;
#17769=EDGE_CURVE ( 'NONE', #7734, #9623, #8173, .T. ) ;
#17932=ADVANCED_FACE ( 'NONE', ( #9383 ), #11219, .F. ) ;
#17987=PRODUCT_DEFINITION_FORMATION_WITH_SPECIFIED_SOURCE ( 'ANY', '', #19255, .NOT_KNOWN. ) ;
#18009=EDGE_LOOP ( 'NONE', ( #12882, #16697, #6329, #18110, #6113, #5528, #9890, #5474 ) ) ;
#18046=DIRECTION ( 'NONE',  ( 0.4627175328665442677, 0.000000000000000000, 0.8865057725575724579 ) ) ;
#18055=ORIENTED_EDGE ( 'NONE', *, *, #5730, .F. ) ;
#18062=PLANE ( 'NONE',  #13874 ) ;
#18083=AXIS2_PLACEMENT_3D ( 'NONE', #9660, #21246, #11390 ) ;
#18110=ORIENTED_EDGE ( 'NONE', *, *, #18733, .T. ) ;
#18245=CARTESIAN_POINT ( 'NONE',  ( 14.09825962131072785, 230.5765313837437418, 49.99999999999999289 ) ) ;
#18248=ORIENTED_EDGE ( 'NONE', *, *, #1000, .T. ) ;
#18325=VERTEX_POINT ( 'NONE', #1544 ) ;
#18343=DIRECTION ( 'NONE',  ( -0.000000000000000000, -0.000000000000000000, 1.000000000000000000 ) ) ;
#18357=ORIENTED_EDGE ( 'NONE', *, *, #11209, .F. ) ;
#18437=ORIENTED_EDGE ( 'NONE', *, *, #15151, .F. ) ;
#18509=DIRECTION ( 'NONE',  ( -2.775557561562891844E-16, 0.000000000000000000, -1.000000000000000000 ) ) ;
#18526=DIRECTION ( 'NONE',  ( 0.000000000000000000, 0.000000000000000000, 1.000000000000000000 ) ) ;
#18591=EDGE_CURVE ( 'NONE', #20328, #2535, #3791, .T. ) ;
#18631=AXIS2_PLACEMENT_3D ( 'NONE', #14820, #8084, #21291 ) ;
#18673=DIRECTION ( 'NONE',  ( 0.000000000000000000, 0.000000000000000000, 1.000000000000000000 ) ) ;
#18733=EDGE_CURVE ( 'NONE', #12668, #18325, #2607, .T. ) ;
#18755=ORIENTED_EDGE ( 'NONE', *, *, #6268, .F. ) ;
#18764=DIRECTION ( 'NONE',  ( 0.000000000000000000, -1.000000000000000000, 0.000000000000000000 ) ) ;
#18807=ORIENTED_EDGE ( 'NONE', *, *, #18733, .F. ) ;
#18826=CARTESIAN_POINT ( 'NONE',  ( 14.09825962131072785, 160.1716627696692683, 49.99999999999999289 ) ) ;
#18917=EDGE_CURVE ( 'NONE', #984, #2721, #14507, .T. ) ;
#18980=AXIS2_PLACEMENT_3D ( 'NONE', #13646, #5197, #12008 ) ;
#19044=CIRCLE ( 'NONE', #12487, 4.000000000000001776 ) ;
#19141=MANIFOLD_SOLID_BREP ( 'Cut-Extrude6[1]', #12097 ) ;
#19149=EDGE_CURVE ( 'NONE', #16828, #6455, #9377, .T. ) ;
#19255=PRODUCT ( 'Ram Linear Way Guides', 'Ram Linear Way Guides', '', ( #16597 ) ) ;
#19278=EDGE_CURVE ( 'NONE', #20328, #18325, #11955, .T. ) ;
#19326=EDGE_CURVE ( 'NONE', #6197, #5267, #8401, .T. ) ;
#19351=DIRECTION ( 'NONE',  ( -0.8865057725575725689, 0.000000000000000000, 0.4627175328665443232 ) ) ;
#19457=AXIS2_PLACEMENT_3D ( 'NONE', #5079, #11458, #4865 ) ;
#19466=DIRECTION ( 'NONE',  ( 0.000000000000000000, -1.000000000000000000, 0.000000000000000000 ) ) ;
#19473=ORIENTED_EDGE ( 'NONE', *, *, #20691, .F. ) ;
#19536=EDGE_CURVE ( 'NONE', #2675, #12300, #9457, .T. ) ;
#19540=DIRECTION ( 'NONE',  ( -1.000000000000000000, 0.000000000000000000, 0.000000000000000000 ) ) ;
#19556=EDGE_LOOP ( 'NONE', ( #5081, #14620, #12983, #191 ) ) ;
#19568=VECTOR ( 'NONE', #11045, 1000.000000000000000 ) ;
#19641=( NAMED_UNIT ( * ) SI_UNIT ( $, .STERADIAN. ) SOLID_ANGLE_UNIT ( ) );
#19670=AXIS2_PLACEMENT_3D ( 'NONE', #10691, #15807, #2386 ) ;
#19676=DIRECTION ( 'NONE',  ( 1.000000000000000000, 0.000000000000000000, 0.000000000000000000 ) ) ;
#19732=ADVANCED_FACE ( 'NONE', ( #6411 ), #4794, .T. ) ;
#19769=VECTOR ( 'NONE', #17157, 1000.000000000000000 ) ;
#19930=CARTESIAN_POINT ( 'NONE',  ( -41.83569717483972994, 230.5765313837437418, 25.00000000000000000 ) ) ;
#19941=EDGE_CURVE ( 'NONE', #2829, #12300, #7021, .T. ) ;
#19971=CARTESIAN_POINT ( 'NONE',  ( 2.416697501590669095, 172.9933428177121471, 45.00000000000000000 ) ) ;
#19973=CARTESIAN_POINT ( 'NONE',  ( 6.416697501590670427, 172.9933428177121471, 49.99999999999999289 ) ) ;
#20009=VERTEX_POINT ( 'NONE', #6817 ) ;
#20020=AXIS2_PLACEMENT_3D ( 'NONE', #12761, #19351, #18046 ) ;
#20095=CARTESIAN_POINT ( 'NONE',  ( -1.025382690249029949, 160.1716627696692683, 25.00000000000000000 ) ) ;
#20212=FACE_OUTER_BOUND ( 'NONE', #1363, .T. ) ;
#20215=PLANE ( 'NONE',  #11961 ) ;
#20271=LINE ( 'NONE', #10303, #13379 ) ;
#20320=DIRECTION ( 'NONE',  ( 0.000000000000000000, 0.000000000000000000, -1.000000000000000000 ) ) ;
#20328=VERTEX_POINT ( 'NONE', #14798 ) ;
#20339=CARTESIAN_POINT ( 'NONE',  ( -41.83569717483972994, 160.1716627696692683, 25.00000000000000000 ) ) ;
#20398=LINE ( 'NONE', #12177, #11643 ) ;
#20431=CARTESIAN_POINT ( 'NONE',  ( 2.416697501590669095, 217.7548513357008630, 45.00000000000000000 ) ) ;
#20550=ORIENTED_EDGE ( 'NONE', *, *, #17488, .T. ) ;
#20567=ORIENTED_EDGE ( 'NONE', *, *, #3150, .F. ) ;
#20691=EDGE_CURVE ( 'NONE', #5267, #6197, #2162, .T. ) ;
#20769=EDGE_LOOP ( 'NONE', ( #3934, #17171 ) ) ;
#20777=APPLICATION_CONTEXT ( 'automotive_design' ) ;
#20802=LINE ( 'NONE', #6073, #19568 ) ;
#20804=DIRECTION ( 'NONE',  ( 0.000000000000000000, 0.000000000000000000, -1.000000000000000000 ) ) ;
#20838=VERTEX_POINT ( 'NONE', #9243 ) ;
#20908=DIRECTION ( 'NONE',  ( 0.000000000000000000, -1.000000000000000000, 0.000000000000000000 ) ) ;
#20917=EDGE_CURVE ( 'NONE', #20009, #2721, #12176, .T. ) ;
#20929=DIRECTION ( 'NONE',  ( -0.000000000000000000, -0.000000000000000000, 1.000000000000000000 ) ) ;
#21065=DIRECTION ( 'NONE',  ( 0.000000000000000000, -1.000000000000000000, 0.000000000000000000 ) ) ;
#21192=PLANE ( 'NONE',  #20020 ) ;
#21246=DIRECTION ( 'NONE',  ( 0.000000000000000000, 0.000000000000000000, -1.000000000000000000 ) ) ;
#21269=( NAMED_UNIT ( * ) PLANE_ANGLE_UNIT ( ) SI_UNIT ( $, .RADIAN. ) );
#21291=DIRECTION ( 'NONE',  ( 1.000000000000000000, 0.000000000000000000, 0.000000000000000000 ) ) ;
#21307=ORIENTED_EDGE ( 'NONE', *, *, #14792, .F. ) ;
#21356=CARTESIAN_POINT ( 'NONE',  ( -54.57497958038185715, 303.6587712403113528, 25.00000000000000000 ) ) ;
#21422=COLOUR_RGB('Sky Blue',0.24,0.69,0.87);
#21423=FILL_AREA_STYLE_COLOUR('',#21422);
#21424=FILL_AREA_STYLE('',(#21423));
#21425=SURFACE_STYLE_FILL_AREA(#21424);
#21426=SURFACE_SIDE_STYLE('',(#21425));
#21427=SURFACE_STYLE_USAGE(.BOTH.,#21426);
#21428=PRESENTATION_STYLE_ASSIGNMENT((#21427));
ENDSEC;
END-ISO-10303-21;
